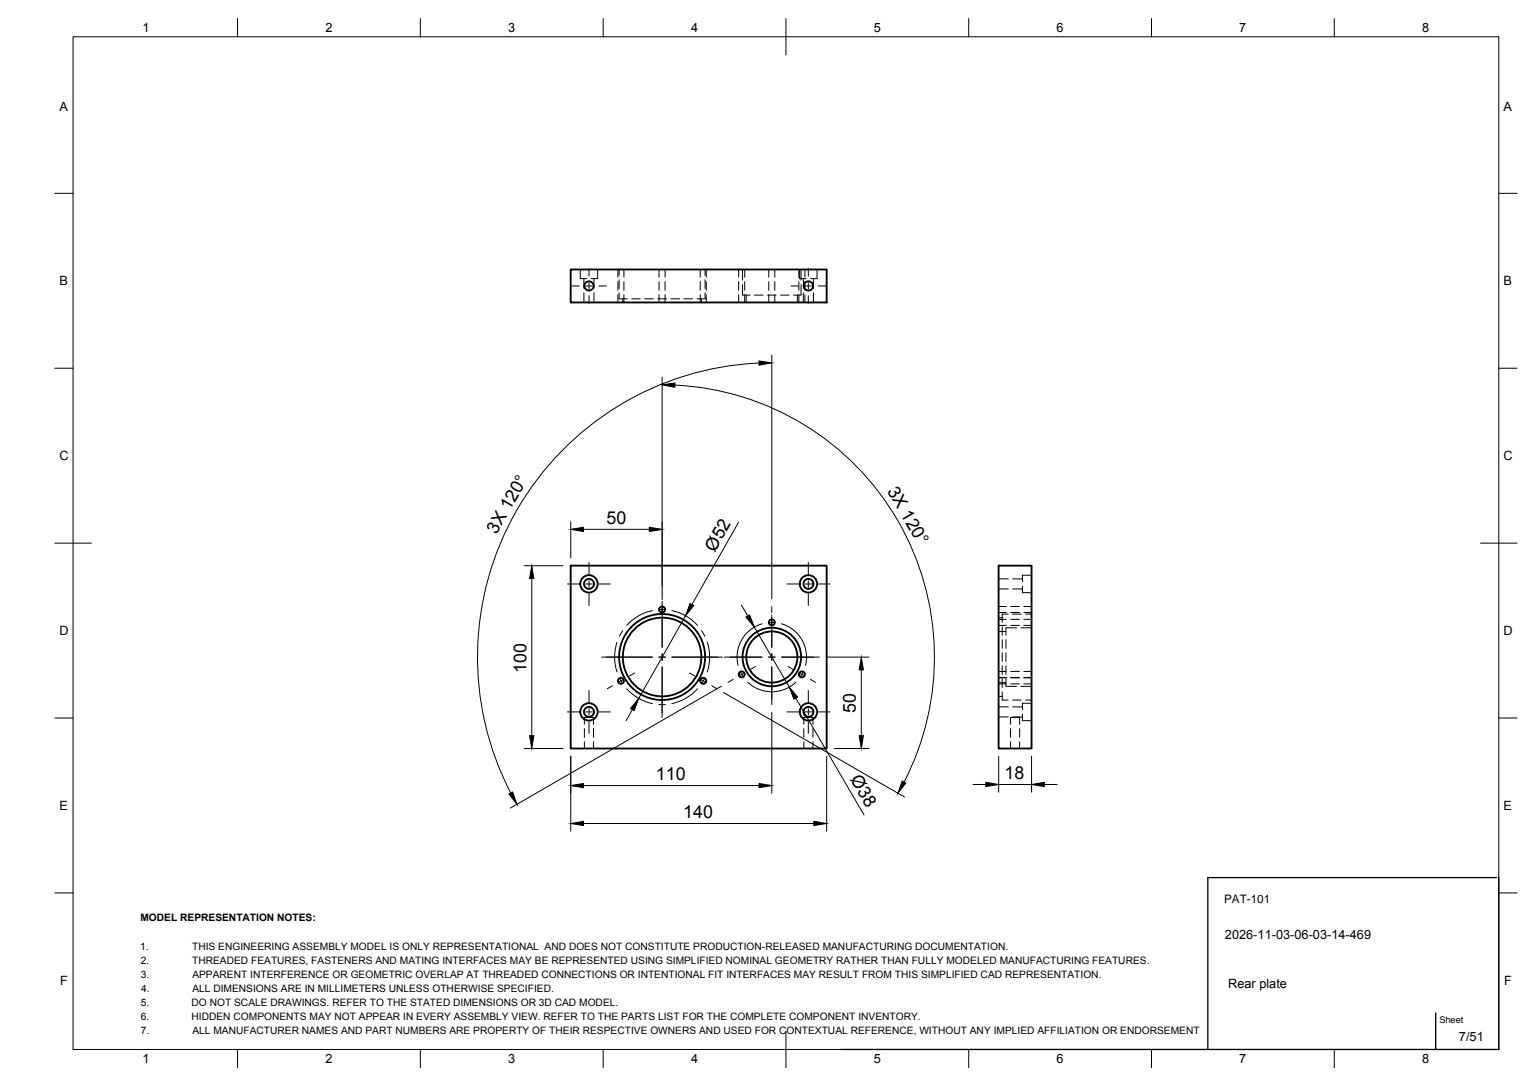
ISO-10303-21;
HEADER;
/* Generated by software containing ST-Developer
 * from STEP Tools, Inc. (www.steptools.com) 
 */

FILE_DESCRIPTION(
/* description */ ('Spur gear reduction stage 2-1 on bearing plates'),
/* implementation_level */ '2;1');

FILE_NAME(
/* name */ 'Rear plate.step',
/* time_stamp */ '2026-10-28T03:22:07-07:00',
/* author */ (''),
/* organization */ (''),
/* preprocessor_version */ 'ST-DEVELOPER v20.2',
/* originating_system */ 'Autodesk Translation Framework v15.17.0.0',
/* authorisation */ '');

FILE_SCHEMA (('AUTOMOTIVE_DESIGN { 1 0 10303 214 3 1 1 }'));
ENDSEC;

DATA;
#10=MECHANICAL_DESIGN_GEOMETRIC_PRESENTATION_REPRESENTATION('',(#949),#53909);
#863=SHAPE_REPRESENTATION_RELATIONSHIP('SRR','None',#54090,#906);
#906=ADVANCED_BREP_SHAPE_REPRESENTATION('',(#1007),#53864);
#949=STYLED_ITEM('',(#54411),#1007);
#1007=MANIFOLD_SOLID_BREP('Body1',#11273);
#1100=FACE_BOUND('',#2243,.T.);
#1101=FACE_BOUND('',#2246,.T.);
#1102=FACE_BOUND('',#2249,.T.);
#1103=FACE_BOUND('',#2252,.T.);
#1104=FACE_BOUND('',#2263,.T.);
#1105=FACE_BOUND('',#2267,.T.);
#1106=FACE_BOUND('',#2270,.T.);
#1107=FACE_BOUND('',#2271,.T.);
#1108=FACE_BOUND('',#2272,.T.);
#1109=FACE_BOUND('',#2273,.T.);
#1110=FACE_BOUND('',#2274,.T.);
#1111=FACE_BOUND('',#2275,.T.);
#1112=FACE_BOUND('',#2276,.T.);
#1113=FACE_BOUND('',#2277,.T.);
#1114=FACE_BOUND('',#2278,.T.);
#1115=FACE_BOUND('',#2279,.T.);
#1116=FACE_BOUND('',#2280,.T.);
#1117=FACE_BOUND('',#2281,.T.);
#1118=FACE_BOUND('',#2284,.T.);
#1119=FACE_BOUND('',#2285,.T.);
#1120=FACE_BOUND('',#2286,.T.);
#1121=FACE_BOUND('',#2287,.T.);
#1122=FACE_BOUND('',#2288,.T.);
#1123=FACE_BOUND('',#2289,.T.);
#1124=FACE_BOUND('',#2290,.T.);
#1125=FACE_BOUND('',#2291,.T.);
#1126=FACE_BOUND('',#2292,.T.);
#1127=FACE_BOUND('',#2293,.T.);
#1128=FACE_BOUND('',#2294,.T.);
#1129=FACE_BOUND('',#2295,.T.);
#1130=FACE_BOUND('',#2299,.T.);
#1131=FACE_BOUND('',#2300,.T.);
#1258=PLANE('',#11924);
#1259=PLANE('',#11929);
#1260=PLANE('',#11934);
#1261=PLANE('',#11939);
#1262=PLANE('',#11952);
#1263=PLANE('',#11956);
#1264=PLANE('',#11960);
#1265=PLANE('',#11967);
#1266=PLANE('',#11971);
#1267=PLANE('',#11972);
#1268=PLANE('',#11973);
#1269=PLANE('',#11974);
#1270=PLANE('',#11975);
#1271=PLANE('',#11976);
#1547=FACE_OUTER_BOUND('',#2235,.T.);
#1548=FACE_OUTER_BOUND('',#2236,.T.);
#1549=FACE_OUTER_BOUND('',#2237,.T.);
#1550=FACE_OUTER_BOUND('',#2238,.T.);
#1551=FACE_OUTER_BOUND('',#2239,.T.);
#1552=FACE_OUTER_BOUND('',#2240,.T.);
#1553=FACE_OUTER_BOUND('',#2241,.T.);
#1554=FACE_OUTER_BOUND('',#2242,.T.);
#1555=FACE_OUTER_BOUND('',#2244,.T.);
#1556=FACE_OUTER_BOUND('',#2245,.T.);
#1557=FACE_OUTER_BOUND('',#2247,.T.);
#1558=FACE_OUTER_BOUND('',#2248,.T.);
#1559=FACE_OUTER_BOUND('',#2250,.T.);
#1560=FACE_OUTER_BOUND('',#2251,.T.);
#1561=FACE_OUTER_BOUND('',#2253,.T.);
#1562=FACE_OUTER_BOUND('',#2254,.T.);
#1563=FACE_OUTER_BOUND('',#2255,.T.);
#1564=FACE_OUTER_BOUND('',#2256,.T.);
#1565=FACE_OUTER_BOUND('',#2257,.T.);
#1566=FACE_OUTER_BOUND('',#2258,.T.);
#1567=FACE_OUTER_BOUND('',#2259,.T.);
#1568=FACE_OUTER_BOUND('',#2260,.T.);
#1569=FACE_OUTER_BOUND('',#2261,.T.);
#1570=FACE_OUTER_BOUND('',#2262,.T.);
#1571=FACE_OUTER_BOUND('',#2264,.T.);
#1572=FACE_OUTER_BOUND('',#2265,.T.);
#1573=FACE_OUTER_BOUND('',#2266,.T.);
#1574=FACE_OUTER_BOUND('',#2268,.T.);
#1575=FACE_OUTER_BOUND('',#2269,.T.);
#1576=FACE_OUTER_BOUND('',#2282,.T.);
#1577=FACE_OUTER_BOUND('',#2283,.T.);
#1578=FACE_OUTER_BOUND('',#2296,.T.);
#1579=FACE_OUTER_BOUND('',#2297,.T.);
#1580=FACE_OUTER_BOUND('',#2298,.T.);
#2235=EDGE_LOOP('',(#7544,#7545,#7546,#7547));
#2236=EDGE_LOOP('',(#7548,#7549,#7550,#7551));
#2237=EDGE_LOOP('',(#7552,#7553,#7554,#7555));
#2238=EDGE_LOOP('',(#7556,#7557,#7558,#7559));
#2239=EDGE_LOOP('',(#7560,#7561,#7562,#7563));
#2240=EDGE_LOOP('',(#7564,#7565,#7566,#7567));
#2241=EDGE_LOOP('',(#7568,#7569,#7570,#7571));
#2242=EDGE_LOOP('',(#7572));
#2243=EDGE_LOOP('',(#7573));
#2244=EDGE_LOOP('',(#7574,#7575,#7576,#7577));
#2245=EDGE_LOOP('',(#7578));
#2246=EDGE_LOOP('',(#7579));
#2247=EDGE_LOOP('',(#7580,#7581,#7582,#7583));
#2248=EDGE_LOOP('',(#7584));
#2249=EDGE_LOOP('',(#7585));
#2250=EDGE_LOOP('',(#7586,#7587,#7588,#7589));
#2251=EDGE_LOOP('',(#7590));
#2252=EDGE_LOOP('',(#7591));
#2253=EDGE_LOOP('',(#7592,#7593,#7594,#7595));
#2254=EDGE_LOOP('',(#7596,#7597,#7598,#7599));
#2255=EDGE_LOOP('',(#7600,#7601,#7602,#7603));
#2256=EDGE_LOOP('',(#7604,#7605,#7606,#7607));
#2257=EDGE_LOOP('',(#7608,#7609,#7610,#7611));
#2258=EDGE_LOOP('',(#7612));
#2259=EDGE_LOOP('',(#7613,#7614,#7615,#7616));
#2260=EDGE_LOOP('',(#7617));
#2261=EDGE_LOOP('',(#7618,#7619,#7620,#7621));
#2262=EDGE_LOOP('',(#7622));
#2263=EDGE_LOOP('',(#7623));
#2264=EDGE_LOOP('',(#7624,#7625,#7626,#7627));
#2265=EDGE_LOOP('',(#7628,#7629,#7630,#7631));
#2266=EDGE_LOOP('',(#7632));
#2267=EDGE_LOOP('',(#7633));
#2268=EDGE_LOOP('',(#7634,#7635,#7636,#7637));
#2269=EDGE_LOOP('',(#7638,#7639,#7640,#7641));
#2270=EDGE_LOOP('',(#7642));
#2271=EDGE_LOOP('',(#7643));
#2272=EDGE_LOOP('',(#7644));
#2273=EDGE_LOOP('',(#7645));
#2274=EDGE_LOOP('',(#7646));
#2275=EDGE_LOOP('',(#7647));
#2276=EDGE_LOOP('',(#7648));
#2277=EDGE_LOOP('',(#7649));
#2278=EDGE_LOOP('',(#7650));
#2279=EDGE_LOOP('',(#7651));
#2280=EDGE_LOOP('',(#7652));
#2281=EDGE_LOOP('',(#7653));
#2282=EDGE_LOOP('',(#7654,#7655,#7656,#7657));
#2283=EDGE_LOOP('',(#7658,#7659,#7660,#7661));
#2284=EDGE_LOOP('',(#7662));
#2285=EDGE_LOOP('',(#7663));
#2286=EDGE_LOOP('',(#7664));
#2287=EDGE_LOOP('',(#7665));
#2288=EDGE_LOOP('',(#7666));
#2289=EDGE_LOOP('',(#7667));
#2290=EDGE_LOOP('',(#7668));
#2291=EDGE_LOOP('',(#7669));
#2292=EDGE_LOOP('',(#7670));
#2293=EDGE_LOOP('',(#7671));
#2294=EDGE_LOOP('',(#7672));
#2295=EDGE_LOOP('',(#7673));
#2296=EDGE_LOOP('',(#7674,#7675,#7676,#7677));
#2297=EDGE_LOOP('',(#7678,#7679,#7680,#7681));
#2298=EDGE_LOOP('',(#7682,#7683,#7684,#7685));
#2299=EDGE_LOOP('',(#7686));
#2300=EDGE_LOOP('',(#7687));
#3025=LINE('',#16188,#3666);
#3026=LINE('',#16194,#3667);
#3027=LINE('',#16200,#3668);
#3028=LINE('',#16206,#3669);
#3029=LINE('',#16212,#3670);
#3030=LINE('',#16218,#3671);
#3031=LINE('',#16224,#3672);
#3032=LINE('',#16233,#3673);
#3033=LINE('',#16242,#3674);
#3034=LINE('',#16251,#3675);
#3035=LINE('',#16259,#3676);
#3036=LINE('',#16263,#3677);
#3037=LINE('',#16267,#3678);
#3038=LINE('',#16271,#3679);
#3039=LINE('',#16276,#3680);
#3040=LINE('',#16283,#3681);
#3041=LINE('',#16290,#3682);
#3042=LINE('',#16298,#3683);
#3043=LINE('',#16303,#3684);
#3044=LINE('',#16311,#3685);
#3045=LINE('',#16315,#3686);
#3046=LINE('',#16317,#3687);
#3047=LINE('',#16319,#3688);
#3048=LINE('',#16320,#3689);
#3049=LINE('',#16323,#3690);
#3050=LINE('',#16325,#3691);
#3051=LINE('',#16326,#3692);
#3052=LINE('',#16329,#3693);
#3053=LINE('',#16331,#3694);
#3054=LINE('',#16332,#3695);
#3055=LINE('',#16334,#3696);
#3056=LINE('',#16335,#3697);
#3666=VECTOR('',#13228,0.165);
#3667=VECTOR('',#13235,0.165);
#3668=VECTOR('',#13242,0.164999999999999);
#3669=VECTOR('',#13249,0.165);
#3670=VECTOR('',#13256,0.165);
#3671=VECTOR('',#13263,0.165);
#3672=VECTOR('',#13270,0.475);
#3673=VECTOR('',#13281,0.475);
#3674=VECTOR('',#13292,0.475);
#3675=VECTOR('',#13303,0.475);
#3676=VECTOR('',#13314,0.275);
#3677=VECTOR('',#13319,0.275);
#3678=VECTOR('',#13324,0.275);
#3679=VECTOR('',#13329,0.275);
#3680=VECTOR('',#13334,0.25);
#3681=VECTOR('',#13343,0.25);
#3682=VECTOR('',#13352,2.35);
#3683=VECTOR('',#13363,2.15);
#3684=VECTOR('',#13368,1.6);
#3685=VECTOR('',#13379,1.4);
#3686=VECTOR('',#13382,1.);
#3687=VECTOR('',#13383,1.);
#3688=VECTOR('',#13384,1.);
#3689=VECTOR('',#13385,1.);
#3690=VECTOR('',#13388,1.);
#3691=VECTOR('',#13389,1.);
#3692=VECTOR('',#13390,1.);
#3693=VECTOR('',#13393,1.);
#3694=VECTOR('',#13394,1.);
#3695=VECTOR('',#13395,1.);
#3696=VECTOR('',#13398,1.);
#3697=VECTOR('',#13399,1.);
#4307=CIRCLE('',#11904,0.165);
#4308=CIRCLE('',#11905,0.165);
#4309=CIRCLE('',#11907,0.165);
#4310=CIRCLE('',#11908,0.165);
#4311=CIRCLE('',#11910,0.164999999999999);
#4312=CIRCLE('',#11911,0.164999999999999);
#4313=CIRCLE('',#11913,0.165);
#4314=CIRCLE('',#11914,0.165);
#4315=CIRCLE('',#11916,0.165);
#4316=CIRCLE('',#11917,0.165);
#4317=CIRCLE('',#11919,0.165);
#4318=CIRCLE('',#11920,0.165);
#4319=CIRCLE('',#11922,0.475);
#4320=CIRCLE('',#11923,0.475);
#4321=CIRCLE('',#11925,0.275);
#4322=CIRCLE('',#11927,0.475);
#4323=CIRCLE('',#11928,0.475);
#4324=CIRCLE('',#11930,0.275);
#4325=CIRCLE('',#11932,0.475);
#4326=CIRCLE('',#11933,0.475);
#4327=CIRCLE('',#11935,0.275);
#4328=CIRCLE('',#11937,0.475);
#4329=CIRCLE('',#11938,0.475);
#4330=CIRCLE('',#11940,0.275);
#4331=CIRCLE('',#11942,0.275);
#4332=CIRCLE('',#11944,0.275);
#4333=CIRCLE('',#11946,0.275);
#4334=CIRCLE('',#11948,0.275);
#4335=CIRCLE('',#11950,0.25);
#4336=CIRCLE('',#11951,0.25);
#4337=CIRCLE('',#11954,0.25);
#4338=CIRCLE('',#11955,0.25);
#4339=CIRCLE('',#11958,2.35);
#4340=CIRCLE('',#11959,2.35);
#4341=CIRCLE('',#11961,2.15);
#4342=CIRCLE('',#11963,2.15);
#4343=CIRCLE('',#11965,1.6);
#4344=CIRCLE('',#11966,1.6);
#4345=CIRCLE('',#11968,1.4);
#4346=CIRCLE('',#11970,1.4);
#4848=VERTEX_POINT('',#16185);
#4849=VERTEX_POINT('',#16187);
#4850=VERTEX_POINT('',#16191);
#4851=VERTEX_POINT('',#16193);
#4852=VERTEX_POINT('',#16197);
#4853=VERTEX_POINT('',#16199);
#4854=VERTEX_POINT('',#16203);
#4855=VERTEX_POINT('',#16205);
#4856=VERTEX_POINT('',#16209);
#4857=VERTEX_POINT('',#16211);
#4858=VERTEX_POINT('',#16215);
#4859=VERTEX_POINT('',#16217);
#4860=VERTEX_POINT('',#16221);
#4861=VERTEX_POINT('',#16223);
#4862=VERTEX_POINT('',#16227);
#4863=VERTEX_POINT('',#16230);
#4864=VERTEX_POINT('',#16232);
#4865=VERTEX_POINT('',#16236);
#4866=VERTEX_POINT('',#16239);
#4867=VERTEX_POINT('',#16241);
#4868=VERTEX_POINT('',#16245);
#4869=VERTEX_POINT('',#16248);
#4870=VERTEX_POINT('',#16250);
#4871=VERTEX_POINT('',#16254);
#4872=VERTEX_POINT('',#16257);
#4873=VERTEX_POINT('',#16261);
#4874=VERTEX_POINT('',#16265);
#4875=VERTEX_POINT('',#16269);
#4876=VERTEX_POINT('',#16273);
#4877=VERTEX_POINT('',#16275);
#4878=VERTEX_POINT('',#16280);
#4879=VERTEX_POINT('',#16282);
#4880=VERTEX_POINT('',#16287);
#4881=VERTEX_POINT('',#16289);
#4882=VERTEX_POINT('',#16293);
#4883=VERTEX_POINT('',#16296);
#4884=VERTEX_POINT('',#16300);
#4885=VERTEX_POINT('',#16302);
#4886=VERTEX_POINT('',#16306);
#4887=VERTEX_POINT('',#16309);
#4888=VERTEX_POINT('',#16313);
#4889=VERTEX_POINT('',#16314);
#4890=VERTEX_POINT('',#16316);
#4891=VERTEX_POINT('',#16318);
#4892=VERTEX_POINT('',#16322);
#4893=VERTEX_POINT('',#16324);
#4894=VERTEX_POINT('',#16328);
#4895=VERTEX_POINT('',#16330);
#5914=EDGE_CURVE('',#4848,#4848,#4307,.T.);
#5915=EDGE_CURVE('',#4848,#4849,#3025,.T.);
#5916=EDGE_CURVE('',#4849,#4849,#4308,.T.);
#5917=EDGE_CURVE('',#4850,#4850,#4309,.T.);
#5918=EDGE_CURVE('',#4850,#4851,#3026,.T.);
#5919=EDGE_CURVE('',#4851,#4851,#4310,.T.);
#5920=EDGE_CURVE('',#4852,#4852,#4311,.T.);
#5921=EDGE_CURVE('',#4852,#4853,#3027,.T.);
#5922=EDGE_CURVE('',#4853,#4853,#4312,.T.);
#5923=EDGE_CURVE('',#4854,#4854,#4313,.T.);
#5924=EDGE_CURVE('',#4854,#4855,#3028,.T.);
#5925=EDGE_CURVE('',#4855,#4855,#4314,.T.);
#5926=EDGE_CURVE('',#4856,#4856,#4315,.T.);
#5927=EDGE_CURVE('',#4856,#4857,#3029,.T.);
#5928=EDGE_CURVE('',#4857,#4857,#4316,.T.);
#5929=EDGE_CURVE('',#4858,#4858,#4317,.T.);
#5930=EDGE_CURVE('',#4858,#4859,#3030,.T.);
#5931=EDGE_CURVE('',#4859,#4859,#4318,.T.);
#5932=EDGE_CURVE('',#4860,#4860,#4319,.T.);
#5933=EDGE_CURVE('',#4860,#4861,#3031,.T.);
#5934=EDGE_CURVE('',#4861,#4861,#4320,.T.);
#5935=EDGE_CURVE('',#4862,#4862,#4321,.T.);
#5936=EDGE_CURVE('',#4863,#4863,#4322,.T.);
#5937=EDGE_CURVE('',#4863,#4864,#3032,.T.);
#5938=EDGE_CURVE('',#4864,#4864,#4323,.T.);
#5939=EDGE_CURVE('',#4865,#4865,#4324,.T.);
#5940=EDGE_CURVE('',#4866,#4866,#4325,.T.);
#5941=EDGE_CURVE('',#4866,#4867,#3033,.T.);
#5942=EDGE_CURVE('',#4867,#4867,#4326,.T.);
#5943=EDGE_CURVE('',#4868,#4868,#4327,.T.);
#5944=EDGE_CURVE('',#4869,#4869,#4328,.T.);
#5945=EDGE_CURVE('',#4869,#4870,#3034,.T.);
#5946=EDGE_CURVE('',#4870,#4870,#4329,.T.);
#5947=EDGE_CURVE('',#4871,#4871,#4330,.T.);
#5948=EDGE_CURVE('',#4872,#4872,#4331,.T.);
#5949=EDGE_CURVE('',#4872,#4862,#3035,.T.);
#5950=EDGE_CURVE('',#4873,#4873,#4332,.T.);
#5951=EDGE_CURVE('',#4873,#4865,#3036,.T.);
#5952=EDGE_CURVE('',#4874,#4874,#4333,.T.);
#5953=EDGE_CURVE('',#4874,#4868,#3037,.T.);
#5954=EDGE_CURVE('',#4875,#4875,#4334,.T.);
#5955=EDGE_CURVE('',#4875,#4871,#3038,.T.);
#5956=EDGE_CURVE('',#4876,#4876,#4335,.T.);
#5957=EDGE_CURVE('',#4876,#4877,#3039,.T.);
#5958=EDGE_CURVE('',#4877,#4877,#4336,.T.);
#5959=EDGE_CURVE('',#4878,#4878,#4337,.T.);
#5960=EDGE_CURVE('',#4878,#4879,#3040,.T.);
#5961=EDGE_CURVE('',#4879,#4879,#4338,.T.);
#5962=EDGE_CURVE('',#4880,#4880,#4339,.T.);
#5963=EDGE_CURVE('',#4880,#4881,#3041,.T.);
#5964=EDGE_CURVE('',#4881,#4881,#4340,.T.);
#5965=EDGE_CURVE('',#4882,#4882,#4341,.T.);
#5966=EDGE_CURVE('',#4883,#4883,#4342,.T.);
#5967=EDGE_CURVE('',#4883,#4882,#3042,.T.);
#5968=EDGE_CURVE('',#4884,#4884,#4343,.T.);
#5969=EDGE_CURVE('',#4884,#4885,#3043,.T.);
#5970=EDGE_CURVE('',#4885,#4885,#4344,.T.);
#5971=EDGE_CURVE('',#4886,#4886,#4345,.T.);
#5972=EDGE_CURVE('',#4887,#4887,#4346,.T.);
#5973=EDGE_CURVE('',#4887,#4886,#3044,.T.);
#5974=EDGE_CURVE('',#4888,#4889,#3045,.T.);
#5975=EDGE_CURVE('',#4889,#4890,#3046,.T.);
#5976=EDGE_CURVE('',#4891,#4890,#3047,.T.);
#5977=EDGE_CURVE('',#4888,#4891,#3048,.T.);
#5978=EDGE_CURVE('',#4892,#4888,#3049,.T.);
#5979=EDGE_CURVE('',#4893,#4891,#3050,.T.);
#5980=EDGE_CURVE('',#4892,#4893,#3051,.T.);
#5981=EDGE_CURVE('',#4894,#4892,#3052,.T.);
#5982=EDGE_CURVE('',#4895,#4893,#3053,.T.);
#5983=EDGE_CURVE('',#4894,#4895,#3054,.T.);
#5984=EDGE_CURVE('',#4889,#4894,#3055,.T.);
#5985=EDGE_CURVE('',#4890,#4895,#3056,.T.);
#7544=ORIENTED_EDGE('',*,*,#5914,.F.);
#7545=ORIENTED_EDGE('',*,*,#5915,.T.);
#7546=ORIENTED_EDGE('',*,*,#5916,.F.);
#7547=ORIENTED_EDGE('',*,*,#5915,.F.);
#7548=ORIENTED_EDGE('',*,*,#5917,.F.);
#7549=ORIENTED_EDGE('',*,*,#5918,.T.);
#7550=ORIENTED_EDGE('',*,*,#5919,.F.);
#7551=ORIENTED_EDGE('',*,*,#5918,.F.);
#7552=ORIENTED_EDGE('',*,*,#5920,.F.);
#7553=ORIENTED_EDGE('',*,*,#5921,.T.);
#7554=ORIENTED_EDGE('',*,*,#5922,.F.);
#7555=ORIENTED_EDGE('',*,*,#5921,.F.);
#7556=ORIENTED_EDGE('',*,*,#5923,.F.);
#7557=ORIENTED_EDGE('',*,*,#5924,.T.);
#7558=ORIENTED_EDGE('',*,*,#5925,.F.);
#7559=ORIENTED_EDGE('',*,*,#5924,.F.);
#7560=ORIENTED_EDGE('',*,*,#5926,.F.);
#7561=ORIENTED_EDGE('',*,*,#5927,.T.);
#7562=ORIENTED_EDGE('',*,*,#5928,.F.);
#7563=ORIENTED_EDGE('',*,*,#5927,.F.);
#7564=ORIENTED_EDGE('',*,*,#5929,.F.);
#7565=ORIENTED_EDGE('',*,*,#5930,.T.);
#7566=ORIENTED_EDGE('',*,*,#5931,.F.);
#7567=ORIENTED_EDGE('',*,*,#5930,.F.);
#7568=ORIENTED_EDGE('',*,*,#5932,.F.);
#7569=ORIENTED_EDGE('',*,*,#5933,.T.);
#7570=ORIENTED_EDGE('',*,*,#5934,.F.);
#7571=ORIENTED_EDGE('',*,*,#5933,.F.);
#7572=ORIENTED_EDGE('',*,*,#5932,.T.);
#7573=ORIENTED_EDGE('',*,*,#5935,.F.);
#7574=ORIENTED_EDGE('',*,*,#5936,.F.);
#7575=ORIENTED_EDGE('',*,*,#5937,.T.);
#7576=ORIENTED_EDGE('',*,*,#5938,.F.);
#7577=ORIENTED_EDGE('',*,*,#5937,.F.);
#7578=ORIENTED_EDGE('',*,*,#5936,.T.);
#7579=ORIENTED_EDGE('',*,*,#5939,.F.);
#7580=ORIENTED_EDGE('',*,*,#5940,.F.);
#7581=ORIENTED_EDGE('',*,*,#5941,.T.);
#7582=ORIENTED_EDGE('',*,*,#5942,.F.);
#7583=ORIENTED_EDGE('',*,*,#5941,.F.);
#7584=ORIENTED_EDGE('',*,*,#5940,.T.);
#7585=ORIENTED_EDGE('',*,*,#5943,.F.);
#7586=ORIENTED_EDGE('',*,*,#5944,.F.);
#7587=ORIENTED_EDGE('',*,*,#5945,.T.);
#7588=ORIENTED_EDGE('',*,*,#5946,.F.);
#7589=ORIENTED_EDGE('',*,*,#5945,.F.);
#7590=ORIENTED_EDGE('',*,*,#5944,.T.);
#7591=ORIENTED_EDGE('',*,*,#5947,.F.);
#7592=ORIENTED_EDGE('',*,*,#5948,.F.);
#7593=ORIENTED_EDGE('',*,*,#5949,.T.);
#7594=ORIENTED_EDGE('',*,*,#5935,.T.);
#7595=ORIENTED_EDGE('',*,*,#5949,.F.);
#7596=ORIENTED_EDGE('',*,*,#5950,.F.);
#7597=ORIENTED_EDGE('',*,*,#5951,.T.);
#7598=ORIENTED_EDGE('',*,*,#5939,.T.);
#7599=ORIENTED_EDGE('',*,*,#5951,.F.);
#7600=ORIENTED_EDGE('',*,*,#5952,.F.);
#7601=ORIENTED_EDGE('',*,*,#5953,.T.);
#7602=ORIENTED_EDGE('',*,*,#5943,.T.);
#7603=ORIENTED_EDGE('',*,*,#5953,.F.);
#7604=ORIENTED_EDGE('',*,*,#5954,.F.);
#7605=ORIENTED_EDGE('',*,*,#5955,.T.);
#7606=ORIENTED_EDGE('',*,*,#5947,.T.);
#7607=ORIENTED_EDGE('',*,*,#5955,.F.);
#7608=ORIENTED_EDGE('',*,*,#5956,.F.);
#7609=ORIENTED_EDGE('',*,*,#5957,.T.);
#7610=ORIENTED_EDGE('',*,*,#5958,.T.);
#7611=ORIENTED_EDGE('',*,*,#5957,.F.);
#7612=ORIENTED_EDGE('',*,*,#5958,.F.);
#7613=ORIENTED_EDGE('',*,*,#5959,.F.);
#7614=ORIENTED_EDGE('',*,*,#5960,.T.);
#7615=ORIENTED_EDGE('',*,*,#5961,.T.);
#7616=ORIENTED_EDGE('',*,*,#5960,.F.);
#7617=ORIENTED_EDGE('',*,*,#5961,.F.);
#7618=ORIENTED_EDGE('',*,*,#5962,.F.);
#7619=ORIENTED_EDGE('',*,*,#5963,.T.);
#7620=ORIENTED_EDGE('',*,*,#5964,.F.);
#7621=ORIENTED_EDGE('',*,*,#5963,.F.);
#7622=ORIENTED_EDGE('',*,*,#5962,.T.);
#7623=ORIENTED_EDGE('',*,*,#5965,.F.);
#7624=ORIENTED_EDGE('',*,*,#5966,.F.);
#7625=ORIENTED_EDGE('',*,*,#5967,.T.);
#7626=ORIENTED_EDGE('',*,*,#5965,.T.);
#7627=ORIENTED_EDGE('',*,*,#5967,.F.);
#7628=ORIENTED_EDGE('',*,*,#5968,.F.);
#7629=ORIENTED_EDGE('',*,*,#5969,.T.);
#7630=ORIENTED_EDGE('',*,*,#5970,.F.);
#7631=ORIENTED_EDGE('',*,*,#5969,.F.);
#7632=ORIENTED_EDGE('',*,*,#5968,.T.);
#7633=ORIENTED_EDGE('',*,*,#5971,.F.);
#7634=ORIENTED_EDGE('',*,*,#5972,.F.);
#7635=ORIENTED_EDGE('',*,*,#5973,.T.);
#7636=ORIENTED_EDGE('',*,*,#5971,.T.);
#7637=ORIENTED_EDGE('',*,*,#5973,.F.);
#7638=ORIENTED_EDGE('',*,*,#5974,.T.);
#7639=ORIENTED_EDGE('',*,*,#5975,.T.);
#7640=ORIENTED_EDGE('',*,*,#5976,.F.);
#7641=ORIENTED_EDGE('',*,*,#5977,.F.);
#7642=ORIENTED_EDGE('',*,*,#5925,.T.);
#7643=ORIENTED_EDGE('',*,*,#5928,.T.);
#7644=ORIENTED_EDGE('',*,*,#5931,.T.);
#7645=ORIENTED_EDGE('',*,*,#5964,.T.);
#7646=ORIENTED_EDGE('',*,*,#5970,.T.);
#7647=ORIENTED_EDGE('',*,*,#5946,.T.);
#7648=ORIENTED_EDGE('',*,*,#5942,.T.);
#7649=ORIENTED_EDGE('',*,*,#5938,.T.);
#7650=ORIENTED_EDGE('',*,*,#5934,.T.);
#7651=ORIENTED_EDGE('',*,*,#5922,.T.);
#7652=ORIENTED_EDGE('',*,*,#5919,.T.);
#7653=ORIENTED_EDGE('',*,*,#5916,.T.);
#7654=ORIENTED_EDGE('',*,*,#5978,.T.);
#7655=ORIENTED_EDGE('',*,*,#5977,.T.);
#7656=ORIENTED_EDGE('',*,*,#5979,.F.);
#7657=ORIENTED_EDGE('',*,*,#5980,.F.);
#7658=ORIENTED_EDGE('',*,*,#5981,.T.);
#7659=ORIENTED_EDGE('',*,*,#5980,.T.);
#7660=ORIENTED_EDGE('',*,*,#5982,.F.);
#7661=ORIENTED_EDGE('',*,*,#5983,.F.);
#7662=ORIENTED_EDGE('',*,*,#5923,.T.);
#7663=ORIENTED_EDGE('',*,*,#5926,.T.);
#7664=ORIENTED_EDGE('',*,*,#5929,.T.);
#7665=ORIENTED_EDGE('',*,*,#5972,.T.);
#7666=ORIENTED_EDGE('',*,*,#5966,.T.);
#7667=ORIENTED_EDGE('',*,*,#5954,.T.);
#7668=ORIENTED_EDGE('',*,*,#5952,.T.);
#7669=ORIENTED_EDGE('',*,*,#5950,.T.);
#7670=ORIENTED_EDGE('',*,*,#5948,.T.);
#7671=ORIENTED_EDGE('',*,*,#5920,.T.);
#7672=ORIENTED_EDGE('',*,*,#5917,.T.);
#7673=ORIENTED_EDGE('',*,*,#5914,.T.);
#7674=ORIENTED_EDGE('',*,*,#5984,.T.);
#7675=ORIENTED_EDGE('',*,*,#5983,.T.);
#7676=ORIENTED_EDGE('',*,*,#5985,.F.);
#7677=ORIENTED_EDGE('',*,*,#5975,.F.);
#7678=ORIENTED_EDGE('',*,*,#5985,.T.);
#7679=ORIENTED_EDGE('',*,*,#5982,.T.);
#7680=ORIENTED_EDGE('',*,*,#5979,.T.);
#7681=ORIENTED_EDGE('',*,*,#5976,.T.);
#7682=ORIENTED_EDGE('',*,*,#5984,.F.);
#7683=ORIENTED_EDGE('',*,*,#5974,.F.);
#7684=ORIENTED_EDGE('',*,*,#5978,.F.);
#7685=ORIENTED_EDGE('',*,*,#5981,.F.);
#7686=ORIENTED_EDGE('',*,*,#5956,.T.);
#7687=ORIENTED_EDGE('',*,*,#5959,.T.);
#10444=CYLINDRICAL_SURFACE('',#11903,0.165);
#10445=CYLINDRICAL_SURFACE('',#11906,0.165);
#10446=CYLINDRICAL_SURFACE('',#11909,0.164999999999999);
#10447=CYLINDRICAL_SURFACE('',#11912,0.165);
#10448=CYLINDRICAL_SURFACE('',#11915,0.165);
#10449=CYLINDRICAL_SURFACE('',#11918,0.165);
#10450=CYLINDRICAL_SURFACE('',#11921,0.475);
#10451=CYLINDRICAL_SURFACE('',#11926,0.475);
#10452=CYLINDRICAL_SURFACE('',#11931,0.475);
#10453=CYLINDRICAL_SURFACE('',#11936,0.475);
#10454=CYLINDRICAL_SURFACE('',#11941,0.275);
#10455=CYLINDRICAL_SURFACE('',#11943,0.275);
#10456=CYLINDRICAL_SURFACE('',#11945,0.275);
#10457=CYLINDRICAL_SURFACE('',#11947,0.275);
#10458=CYLINDRICAL_SURFACE('',#11949,0.25);
#10459=CYLINDRICAL_SURFACE('',#11953,0.25);
#10460=CYLINDRICAL_SURFACE('',#11957,2.35);
#10461=CYLINDRICAL_SURFACE('',#11962,2.15);
#10462=CYLINDRICAL_SURFACE('',#11964,1.6);
#10463=CYLINDRICAL_SURFACE('',#11969,1.4);
#10667=ADVANCED_FACE('',(#1547),#10444,.F.);
#10668=ADVANCED_FACE('',(#1548),#10445,.F.);
#10669=ADVANCED_FACE('',(#1549),#10446,.F.);
#10670=ADVANCED_FACE('',(#1550),#10447,.F.);
#10671=ADVANCED_FACE('',(#1551),#10448,.F.);
#10672=ADVANCED_FACE('',(#1552),#10449,.F.);
#10673=ADVANCED_FACE('',(#1553),#10450,.F.);
#10674=ADVANCED_FACE('',(#1554,#1100),#1258,.T.);
#10675=ADVANCED_FACE('',(#1555),#10451,.F.);
#10676=ADVANCED_FACE('',(#1556,#1101),#1259,.T.);
#10677=ADVANCED_FACE('',(#1557),#10452,.F.);
#10678=ADVANCED_FACE('',(#1558,#1102),#1260,.T.);
#10679=ADVANCED_FACE('',(#1559),#10453,.F.);
#10680=ADVANCED_FACE('',(#1560,#1103),#1261,.T.);
#10681=ADVANCED_FACE('',(#1561),#10454,.F.);
#10682=ADVANCED_FACE('',(#1562),#10455,.F.);
#10683=ADVANCED_FACE('',(#1563),#10456,.F.);
#10684=ADVANCED_FACE('',(#1564),#10457,.F.);
#10685=ADVANCED_FACE('',(#1565),#10458,.F.);
#10686=ADVANCED_FACE('',(#1566),#1262,.F.);
#10687=ADVANCED_FACE('',(#1567),#10459,.F.);
#10688=ADVANCED_FACE('',(#1568),#1263,.F.);
#10689=ADVANCED_FACE('',(#1569),#10460,.F.);
#10690=ADVANCED_FACE('',(#1570,#1104),#1264,.T.);
#10691=ADVANCED_FACE('',(#1571),#10461,.F.);
#10692=ADVANCED_FACE('',(#1572),#10462,.F.);
#10693=ADVANCED_FACE('',(#1573,#1105),#1265,.T.);
#10694=ADVANCED_FACE('',(#1574),#10463,.F.);
#10695=ADVANCED_FACE('',(#1575,#1106,#1107,#1108,#1109,#1110,#1111,#1112,
#1113,#1114,#1115,#1116,#1117),#1266,.T.);
#10696=ADVANCED_FACE('',(#1576),#1267,.T.);
#10697=ADVANCED_FACE('',(#1577,#1118,#1119,#1120,#1121,#1122,#1123,#1124,
#1125,#1126,#1127,#1128,#1129),#1268,.T.);
#10698=ADVANCED_FACE('',(#1578),#1269,.T.);
#10699=ADVANCED_FACE('',(#1579),#1270,.T.);
#10700=ADVANCED_FACE('',(#1580,#1130,#1131),#1271,.F.);
#11273=CLOSED_SHELL('',(#10667,#10668,#10669,#10670,#10671,#10672,#10673,
#10674,#10675,#10676,#10677,#10678,#10679,#10680,#10681,#10682,#10683,#10684,
#10685,#10686,#10687,#10688,#10689,#10690,#10691,#10692,#10693,#10694,#10695,
#10696,#10697,#10698,#10699,#10700));
#11902=AXIS2_PLACEMENT_3D('',#16183,#13222,#13223);
#11903=AXIS2_PLACEMENT_3D('',#16184,#13224,#13225);
#11904=AXIS2_PLACEMENT_3D('',#16186,#13226,#13227);
#11905=AXIS2_PLACEMENT_3D('',#16189,#13229,#13230);
#11906=AXIS2_PLACEMENT_3D('',#16190,#13231,#13232);
#11907=AXIS2_PLACEMENT_3D('',#16192,#13233,#13234);
#11908=AXIS2_PLACEMENT_3D('',#16195,#13236,#13237);
#11909=AXIS2_PLACEMENT_3D('',#16196,#13238,#13239);
#11910=AXIS2_PLACEMENT_3D('',#16198,#13240,#13241);
#11911=AXIS2_PLACEMENT_3D('',#16201,#13243,#13244);
#11912=AXIS2_PLACEMENT_3D('',#16202,#13245,#13246);
#11913=AXIS2_PLACEMENT_3D('',#16204,#13247,#13248);
#11914=AXIS2_PLACEMENT_3D('',#16207,#13250,#13251);
#11915=AXIS2_PLACEMENT_3D('',#16208,#13252,#13253);
#11916=AXIS2_PLACEMENT_3D('',#16210,#13254,#13255);
#11917=AXIS2_PLACEMENT_3D('',#16213,#13257,#13258);
#11918=AXIS2_PLACEMENT_3D('',#16214,#13259,#13260);
#11919=AXIS2_PLACEMENT_3D('',#16216,#13261,#13262);
#11920=AXIS2_PLACEMENT_3D('',#16219,#13264,#13265);
#11921=AXIS2_PLACEMENT_3D('',#16220,#13266,#13267);
#11922=AXIS2_PLACEMENT_3D('',#16222,#13268,#13269);
#11923=AXIS2_PLACEMENT_3D('',#16225,#13271,#13272);
#11924=AXIS2_PLACEMENT_3D('',#16226,#13273,#13274);
#11925=AXIS2_PLACEMENT_3D('',#16228,#13275,#13276);
#11926=AXIS2_PLACEMENT_3D('',#16229,#13277,#13278);
#11927=AXIS2_PLACEMENT_3D('',#16231,#13279,#13280);
#11928=AXIS2_PLACEMENT_3D('',#16234,#13282,#13283);
#11929=AXIS2_PLACEMENT_3D('',#16235,#13284,#13285);
#11930=AXIS2_PLACEMENT_3D('',#16237,#13286,#13287);
#11931=AXIS2_PLACEMENT_3D('',#16238,#13288,#13289);
#11932=AXIS2_PLACEMENT_3D('',#16240,#13290,#13291);
#11933=AXIS2_PLACEMENT_3D('',#16243,#13293,#13294);
#11934=AXIS2_PLACEMENT_3D('',#16244,#13295,#13296);
#11935=AXIS2_PLACEMENT_3D('',#16246,#13297,#13298);
#11936=AXIS2_PLACEMENT_3D('',#16247,#13299,#13300);
#11937=AXIS2_PLACEMENT_3D('',#16249,#13301,#13302);
#11938=AXIS2_PLACEMENT_3D('',#16252,#13304,#13305);
#11939=AXIS2_PLACEMENT_3D('',#16253,#13306,#13307);
#11940=AXIS2_PLACEMENT_3D('',#16255,#13308,#13309);
#11941=AXIS2_PLACEMENT_3D('',#16256,#13310,#13311);
#11942=AXIS2_PLACEMENT_3D('',#16258,#13312,#13313);
#11943=AXIS2_PLACEMENT_3D('',#16260,#13315,#13316);
#11944=AXIS2_PLACEMENT_3D('',#16262,#13317,#13318);
#11945=AXIS2_PLACEMENT_3D('',#16264,#13320,#13321);
#11946=AXIS2_PLACEMENT_3D('',#16266,#13322,#13323);
#11947=AXIS2_PLACEMENT_3D('',#16268,#13325,#13326);
#11948=AXIS2_PLACEMENT_3D('',#16270,#13327,#13328);
#11949=AXIS2_PLACEMENT_3D('',#16272,#13330,#13331);
#11950=AXIS2_PLACEMENT_3D('',#16274,#13332,#13333);
#11951=AXIS2_PLACEMENT_3D('',#16277,#13335,#13336);
#11952=AXIS2_PLACEMENT_3D('',#16278,#13337,#13338);
#11953=AXIS2_PLACEMENT_3D('',#16279,#13339,#13340);
#11954=AXIS2_PLACEMENT_3D('',#16281,#13341,#13342);
#11955=AXIS2_PLACEMENT_3D('',#16284,#13344,#13345);
#11956=AXIS2_PLACEMENT_3D('',#16285,#13346,#13347);
#11957=AXIS2_PLACEMENT_3D('',#16286,#13348,#13349);
#11958=AXIS2_PLACEMENT_3D('',#16288,#13350,#13351);
#11959=AXIS2_PLACEMENT_3D('',#16291,#13353,#13354);
#11960=AXIS2_PLACEMENT_3D('',#16292,#13355,#13356);
#11961=AXIS2_PLACEMENT_3D('',#16294,#13357,#13358);
#11962=AXIS2_PLACEMENT_3D('',#16295,#13359,#13360);
#11963=AXIS2_PLACEMENT_3D('',#16297,#13361,#13362);
#11964=AXIS2_PLACEMENT_3D('',#16299,#13364,#13365);
#11965=AXIS2_PLACEMENT_3D('',#16301,#13366,#13367);
#11966=AXIS2_PLACEMENT_3D('',#16304,#13369,#13370);
#11967=AXIS2_PLACEMENT_3D('',#16305,#13371,#13372);
#11968=AXIS2_PLACEMENT_3D('',#16307,#13373,#13374);
#11969=AXIS2_PLACEMENT_3D('',#16308,#13375,#13376);
#11970=AXIS2_PLACEMENT_3D('',#16310,#13377,#13378);
#11971=AXIS2_PLACEMENT_3D('',#16312,#13380,#13381);
#11972=AXIS2_PLACEMENT_3D('',#16321,#13386,#13387);
#11973=AXIS2_PLACEMENT_3D('',#16327,#13391,#13392);
#11974=AXIS2_PLACEMENT_3D('',#16333,#13396,#13397);
#11975=AXIS2_PLACEMENT_3D('',#16336,#13400,#13401);
#11976=AXIS2_PLACEMENT_3D('',#16337,#13402,#13403);
#13222=DIRECTION('axis',(0.,0.,1.));
#13223=DIRECTION('refdir',(1.,0.,0.));
#13224=DIRECTION('center_axis',(0.,1.,0.));
#13225=DIRECTION('ref_axis',(1.,0.,0.));
#13226=DIRECTION('center_axis',(0.,1.,0.));
#13227=DIRECTION('ref_axis',(1.,0.,0.));
#13228=DIRECTION('',(0.,1.,0.));
#13229=DIRECTION('center_axis',(0.,-1.,0.));
#13230=DIRECTION('ref_axis',(1.,0.,0.));
#13231=DIRECTION('center_axis',(0.,1.,0.));
#13232=DIRECTION('ref_axis',(1.,0.,0.));
#13233=DIRECTION('center_axis',(0.,1.,0.));
#13234=DIRECTION('ref_axis',(1.,0.,0.));
#13235=DIRECTION('',(0.,1.,0.));
#13236=DIRECTION('center_axis',(0.,-1.,0.));
#13237=DIRECTION('ref_axis',(1.,0.,0.));
#13238=DIRECTION('center_axis',(0.,1.,0.));
#13239=DIRECTION('ref_axis',(1.,0.,0.));
#13240=DIRECTION('center_axis',(0.,1.,0.));
#13241=DIRECTION('ref_axis',(1.,0.,0.));
#13242=DIRECTION('',(0.,1.,0.));
#13243=DIRECTION('center_axis',(0.,-1.,0.));
#13244=DIRECTION('ref_axis',(1.,0.,0.));
#13245=DIRECTION('center_axis',(0.,1.,0.));
#13246=DIRECTION('ref_axis',(1.,0.,0.));
#13247=DIRECTION('center_axis',(0.,1.,0.));
#13248=DIRECTION('ref_axis',(1.,0.,0.));
#13249=DIRECTION('',(0.,1.,0.));
#13250=DIRECTION('center_axis',(0.,-1.,0.));
#13251=DIRECTION('ref_axis',(1.,0.,0.));
#13252=DIRECTION('center_axis',(0.,1.,0.));
#13253=DIRECTION('ref_axis',(1.,0.,0.));
#13254=DIRECTION('center_axis',(0.,1.,0.));
#13255=DIRECTION('ref_axis',(1.,0.,0.));
#13256=DIRECTION('',(0.,1.,0.));
#13257=DIRECTION('center_axis',(0.,-1.,0.));
#13258=DIRECTION('ref_axis',(1.,0.,0.));
#13259=DIRECTION('center_axis',(0.,1.,0.));
#13260=DIRECTION('ref_axis',(1.,0.,0.));
#13261=DIRECTION('center_axis',(0.,1.,0.));
#13262=DIRECTION('ref_axis',(1.,0.,0.));
#13263=DIRECTION('',(0.,1.,0.));
#13264=DIRECTION('center_axis',(0.,-1.,0.));
#13265=DIRECTION('ref_axis',(1.,0.,0.));
#13266=DIRECTION('center_axis',(0.,1.,0.));
#13267=DIRECTION('ref_axis',(1.,0.,0.));
#13268=DIRECTION('center_axis',(0.,1.,0.));
#13269=DIRECTION('ref_axis',(1.,0.,0.));
#13270=DIRECTION('',(0.,1.,0.));
#13271=DIRECTION('center_axis',(0.,-1.,0.));
#13272=DIRECTION('ref_axis',(1.,0.,0.));
#13273=DIRECTION('center_axis',(0.,1.,0.));
#13274=DIRECTION('ref_axis',(1.,0.,0.));
#13275=DIRECTION('center_axis',(0.,1.,0.));
#13276=DIRECTION('ref_axis',(1.,0.,0.));
#13277=DIRECTION('center_axis',(0.,1.,0.));
#13278=DIRECTION('ref_axis',(1.,0.,0.));
#13279=DIRECTION('center_axis',(0.,1.,0.));
#13280=DIRECTION('ref_axis',(1.,0.,0.));
#13281=DIRECTION('',(0.,1.,0.));
#13282=DIRECTION('center_axis',(0.,-1.,0.));
#13283=DIRECTION('ref_axis',(1.,0.,0.));
#13284=DIRECTION('center_axis',(0.,1.,0.));
#13285=DIRECTION('ref_axis',(1.,0.,0.));
#13286=DIRECTION('center_axis',(0.,1.,0.));
#13287=DIRECTION('ref_axis',(1.,0.,0.));
#13288=DIRECTION('center_axis',(0.,1.,0.));
#13289=DIRECTION('ref_axis',(1.,0.,0.));
#13290=DIRECTION('center_axis',(0.,1.,0.));
#13291=DIRECTION('ref_axis',(1.,0.,0.));
#13292=DIRECTION('',(0.,1.,0.));
#13293=DIRECTION('center_axis',(0.,-1.,0.));
#13294=DIRECTION('ref_axis',(1.,0.,0.));
#13295=DIRECTION('center_axis',(0.,1.,0.));
#13296=DIRECTION('ref_axis',(1.,0.,0.));
#13297=DIRECTION('center_axis',(0.,1.,0.));
#13298=DIRECTION('ref_axis',(1.,0.,0.));
#13299=DIRECTION('center_axis',(0.,1.,0.));
#13300=DIRECTION('ref_axis',(1.,0.,0.));
#13301=DIRECTION('center_axis',(0.,1.,0.));
#13302=DIRECTION('ref_axis',(1.,0.,0.));
#13303=DIRECTION('',(0.,1.,0.));
#13304=DIRECTION('center_axis',(0.,-1.,0.));
#13305=DIRECTION('ref_axis',(1.,0.,0.));
#13306=DIRECTION('center_axis',(0.,1.,0.));
#13307=DIRECTION('ref_axis',(1.,0.,0.));
#13308=DIRECTION('center_axis',(0.,1.,0.));
#13309=DIRECTION('ref_axis',(1.,0.,0.));
#13310=DIRECTION('center_axis',(0.,1.,0.));
#13311=DIRECTION('ref_axis',(1.,0.,0.));
#13312=DIRECTION('center_axis',(0.,1.,0.));
#13313=DIRECTION('ref_axis',(1.,0.,0.));
#13314=DIRECTION('',(0.,1.,0.));
#13315=DIRECTION('center_axis',(0.,1.,0.));
#13316=DIRECTION('ref_axis',(1.,0.,0.));
#13317=DIRECTION('center_axis',(0.,1.,0.));
#13318=DIRECTION('ref_axis',(1.,0.,0.));
#13319=DIRECTION('',(0.,1.,0.));
#13320=DIRECTION('center_axis',(0.,1.,0.));
#13321=DIRECTION('ref_axis',(1.,0.,0.));
#13322=DIRECTION('center_axis',(0.,1.,0.));
#13323=DIRECTION('ref_axis',(1.,0.,0.));
#13324=DIRECTION('',(0.,1.,0.));
#13325=DIRECTION('center_axis',(0.,1.,0.));
#13326=DIRECTION('ref_axis',(1.,0.,0.));
#13327=DIRECTION('center_axis',(0.,1.,0.));
#13328=DIRECTION('ref_axis',(1.,0.,0.));
#13329=DIRECTION('',(0.,1.,0.));
#13330=DIRECTION('center_axis',(0.,0.,1.));
#13331=DIRECTION('ref_axis',(1.,0.,0.));
#13332=DIRECTION('center_axis',(0.,0.,1.));
#13333=DIRECTION('ref_axis',(1.,0.,0.));
#13334=DIRECTION('',(0.,0.,1.));
#13335=DIRECTION('center_axis',(0.,0.,1.));
#13336=DIRECTION('ref_axis',(1.,0.,0.));
#13337=DIRECTION('center_axis',(0.,0.,1.));
#13338=DIRECTION('ref_axis',(1.,0.,0.));
#13339=DIRECTION('center_axis',(0.,0.,1.));
#13340=DIRECTION('ref_axis',(1.,0.,0.));
#13341=DIRECTION('center_axis',(0.,0.,1.));
#13342=DIRECTION('ref_axis',(1.,0.,0.));
#13343=DIRECTION('',(0.,0.,1.));
#13344=DIRECTION('center_axis',(0.,0.,1.));
#13345=DIRECTION('ref_axis',(1.,0.,0.));
#13346=DIRECTION('center_axis',(0.,0.,1.));
#13347=DIRECTION('ref_axis',(1.,0.,0.));
#13348=DIRECTION('center_axis',(0.,1.,0.));
#13349=DIRECTION('ref_axis',(1.,0.,0.));
#13350=DIRECTION('center_axis',(0.,1.,0.));
#13351=DIRECTION('ref_axis',(1.,0.,0.));
#13352=DIRECTION('',(0.,1.,0.));
#13353=DIRECTION('center_axis',(0.,-1.,0.));
#13354=DIRECTION('ref_axis',(1.,0.,0.));
#13355=DIRECTION('center_axis',(0.,1.,0.));
#13356=DIRECTION('ref_axis',(1.,0.,0.));
#13357=DIRECTION('center_axis',(0.,1.,0.));
#13358=DIRECTION('ref_axis',(1.,0.,0.));
#13359=DIRECTION('center_axis',(0.,1.,0.));
#13360=DIRECTION('ref_axis',(1.,0.,0.));
#13361=DIRECTION('center_axis',(0.,1.,0.));
#13362=DIRECTION('ref_axis',(1.,0.,0.));
#13363=DIRECTION('',(0.,1.,0.));
#13364=DIRECTION('center_axis',(0.,1.,0.));
#13365=DIRECTION('ref_axis',(1.,0.,0.));
#13366=DIRECTION('center_axis',(0.,1.,0.));
#13367=DIRECTION('ref_axis',(1.,0.,0.));
#13368=DIRECTION('',(0.,1.,0.));
#13369=DIRECTION('center_axis',(0.,-1.,0.));
#13370=DIRECTION('ref_axis',(1.,0.,0.));
#13371=DIRECTION('center_axis',(0.,1.,0.));
#13372=DIRECTION('ref_axis',(1.,0.,0.));
#13373=DIRECTION('center_axis',(0.,1.,0.));
#13374=DIRECTION('ref_axis',(1.,0.,0.));
#13375=DIRECTION('center_axis',(0.,1.,0.));
#13376=DIRECTION('ref_axis',(1.,0.,0.));
#13377=DIRECTION('center_axis',(0.,1.,0.));
#13378=DIRECTION('ref_axis',(1.,0.,0.));
#13379=DIRECTION('',(0.,1.,0.));
#13380=DIRECTION('center_axis',(0.,1.,0.));
#13381=DIRECTION('ref_axis',(-1.,0.,0.));
#13382=DIRECTION('',(-1.,0.,0.));
#13383=DIRECTION('',(0.,0.,1.));
#13384=DIRECTION('',(-1.,0.,0.));
#13385=DIRECTION('',(0.,0.,1.));
#13386=DIRECTION('center_axis',(1.,0.,0.));
#13387=DIRECTION('ref_axis',(0.,1.,0.));
#13388=DIRECTION('',(0.,1.,0.));
#13389=DIRECTION('',(0.,1.,0.));
#13390=DIRECTION('',(0.,0.,1.));
#13391=DIRECTION('center_axis',(0.,-1.,0.));
#13392=DIRECTION('ref_axis',(1.,0.,0.));
#13393=DIRECTION('',(1.,0.,0.));
#13394=DIRECTION('',(1.,0.,0.));
#13395=DIRECTION('',(0.,0.,1.));
#13396=DIRECTION('center_axis',(-1.,0.,0.));
#13397=DIRECTION('ref_axis',(0.,-1.,0.));
#13398=DIRECTION('',(0.,-1.,0.));
#13399=DIRECTION('',(0.,-1.,0.));
#13400=DIRECTION('center_axis',(0.,0.,1.));
#13401=DIRECTION('ref_axis',(1.,0.,0.));
#13402=DIRECTION('center_axis',(0.,0.,1.));
#13403=DIRECTION('ref_axis',(1.,0.,0.));
#16183=CARTESIAN_POINT('',(0.,0.,0.));
#16184=CARTESIAN_POINT('Origin',(6.,2.5,7.6));
#16185=CARTESIAN_POINT('',(5.835,2.6,7.6));
#16186=CARTESIAN_POINT('Origin',(6.,2.6,7.6));
#16187=CARTESIAN_POINT('',(5.835,4.4,7.6));
#16188=CARTESIAN_POINT('',(5.835,2.5,7.6));
#16189=CARTESIAN_POINT('Origin',(6.,4.4,7.6));
#16190=CARTESIAN_POINT('Origin',(3.74833395016046,2.5,3.7));
#16191=CARTESIAN_POINT('',(3.58333395016046,2.6,3.7));
#16192=CARTESIAN_POINT('Origin',(3.74833395016046,2.6,3.7));
#16193=CARTESIAN_POINT('',(3.58333395016046,4.4,3.7));
#16194=CARTESIAN_POINT('',(3.58333395016046,2.5,3.7));
#16195=CARTESIAN_POINT('Origin',(3.74833395016046,4.4,3.7));
#16196=CARTESIAN_POINT('Origin',(8.25166604983954,2.5,3.7));
#16197=CARTESIAN_POINT('',(8.08666604983954,2.6,3.7));
#16198=CARTESIAN_POINT('Origin',(8.25166604983954,2.6,3.7));
#16199=CARTESIAN_POINT('',(8.08666604983954,4.4,3.7));
#16200=CARTESIAN_POINT('',(8.08666604983954,2.5,3.7));
#16201=CARTESIAN_POINT('Origin',(8.25166604983954,4.4,3.7));
#16202=CARTESIAN_POINT('Origin',(1.16341445918999E-16,2.5,6.9));
#16203=CARTESIAN_POINT('',(-0.165,2.6,6.9));
#16204=CARTESIAN_POINT('Origin',(1.16341445918999E-16,2.6,6.9));
#16205=CARTESIAN_POINT('',(-0.165,4.4,6.9));
#16206=CARTESIAN_POINT('',(-0.165,2.5,6.9));
#16207=CARTESIAN_POINT('Origin',(1.16341445918999E-16,4.4,6.9));
#16208=CARTESIAN_POINT('Origin',(-1.64544826719043,2.5,4.05));
#16209=CARTESIAN_POINT('',(-1.81044826719043,2.6,4.05));
#16210=CARTESIAN_POINT('Origin',(-1.64544826719043,2.6,4.05));
#16211=CARTESIAN_POINT('',(-1.81044826719043,4.4,4.05));
#16212=CARTESIAN_POINT('',(-1.81044826719043,2.5,4.05));
#16213=CARTESIAN_POINT('Origin',(-1.64544826719043,4.4,4.05));
#16214=CARTESIAN_POINT('Origin',(1.64544826719043,2.5,4.05));
#16215=CARTESIAN_POINT('',(1.48044826719043,2.6,4.05));
#16216=CARTESIAN_POINT('Origin',(1.64544826719043,2.6,4.05));
#16217=CARTESIAN_POINT('',(1.48044826719043,4.4,4.05));
#16218=CARTESIAN_POINT('',(1.48044826719043,2.5,4.05));
#16219=CARTESIAN_POINT('Origin',(1.64544826719043,4.4,4.05));
#16220=CARTESIAN_POINT('Origin',(10.,3.9,2.));
#16221=CARTESIAN_POINT('',(9.525,3.9,2.));
#16222=CARTESIAN_POINT('Origin',(10.,3.9,2.));
#16223=CARTESIAN_POINT('',(9.525,4.4,2.));
#16224=CARTESIAN_POINT('',(9.525,3.9,2.));
#16225=CARTESIAN_POINT('Origin',(10.,4.4,2.));
#16226=CARTESIAN_POINT('Origin',(10.,3.9,2.));
#16227=CARTESIAN_POINT('',(9.725,3.9,2.));
#16228=CARTESIAN_POINT('Origin',(10.,3.9,2.));
#16229=CARTESIAN_POINT('Origin',(-2.,3.9,9.));
#16230=CARTESIAN_POINT('',(-2.475,3.9,9.));
#16231=CARTESIAN_POINT('Origin',(-2.,3.9,9.));
#16232=CARTESIAN_POINT('',(-2.475,4.4,9.));
#16233=CARTESIAN_POINT('',(-2.475,3.9,9.));
#16234=CARTESIAN_POINT('Origin',(-2.,4.4,9.));
#16235=CARTESIAN_POINT('Origin',(-2.,3.9,9.));
#16236=CARTESIAN_POINT('',(-2.275,3.9,9.));
#16237=CARTESIAN_POINT('Origin',(-2.,3.9,9.));
#16238=CARTESIAN_POINT('Origin',(-2.,3.9,2.));
#16239=CARTESIAN_POINT('',(-2.475,3.9,2.));
#16240=CARTESIAN_POINT('Origin',(-2.,3.9,2.));
#16241=CARTESIAN_POINT('',(-2.475,4.4,2.));
#16242=CARTESIAN_POINT('',(-2.475,3.9,2.));
#16243=CARTESIAN_POINT('Origin',(-2.,4.4,2.));
#16244=CARTESIAN_POINT('Origin',(-2.,3.9,2.));
#16245=CARTESIAN_POINT('',(-2.275,3.9,2.));
#16246=CARTESIAN_POINT('Origin',(-2.,3.9,2.));
#16247=CARTESIAN_POINT('Origin',(10.,3.9,9.));
#16248=CARTESIAN_POINT('',(9.525,3.9,9.));
#16249=CARTESIAN_POINT('Origin',(10.,3.9,9.));
#16250=CARTESIAN_POINT('',(9.525,4.4,9.));
#16251=CARTESIAN_POINT('',(9.525,3.9,9.));
#16252=CARTESIAN_POINT('Origin',(10.,4.4,9.));
#16253=CARTESIAN_POINT('Origin',(10.,3.9,9.));
#16254=CARTESIAN_POINT('',(9.725,3.9,9.));
#16255=CARTESIAN_POINT('Origin',(10.,3.9,9.));
#16256=CARTESIAN_POINT('Origin',(10.,2.5,2.));
#16257=CARTESIAN_POINT('',(9.725,2.6,2.));
#16258=CARTESIAN_POINT('Origin',(10.,2.6,2.));
#16259=CARTESIAN_POINT('',(9.725,2.5,2.));
#16260=CARTESIAN_POINT('Origin',(-2.,2.5,9.));
#16261=CARTESIAN_POINT('',(-2.275,2.6,9.));
#16262=CARTESIAN_POINT('Origin',(-2.,2.6,9.));
#16263=CARTESIAN_POINT('',(-2.275,2.5,9.));
#16264=CARTESIAN_POINT('Origin',(-2.,2.5,2.));
#16265=CARTESIAN_POINT('',(-2.275,2.6,2.));
#16266=CARTESIAN_POINT('Origin',(-2.,2.6,2.));
#16267=CARTESIAN_POINT('',(-2.275,2.5,2.));
#16268=CARTESIAN_POINT('Origin',(10.,2.5,9.));
#16269=CARTESIAN_POINT('',(9.725,2.6,9.));
#16270=CARTESIAN_POINT('Origin',(10.,2.6,9.));
#16271=CARTESIAN_POINT('',(9.725,2.5,9.));
#16272=CARTESIAN_POINT('Origin',(10.,3.5,-0.1));
#16273=CARTESIAN_POINT('',(9.75,3.5,0.));
#16274=CARTESIAN_POINT('Origin',(10.,3.5,0.));
#16275=CARTESIAN_POINT('',(9.75,3.5,1.7));
#16276=CARTESIAN_POINT('',(9.75,3.5,-0.1));
#16277=CARTESIAN_POINT('Origin',(10.,3.5,1.7));
#16278=CARTESIAN_POINT('Origin',(10.,3.5,1.7));
#16279=CARTESIAN_POINT('Origin',(-2.,3.5,-0.1));
#16280=CARTESIAN_POINT('',(-2.25,3.5,0.));
#16281=CARTESIAN_POINT('Origin',(-2.,3.5,0.));
#16282=CARTESIAN_POINT('',(-2.25,3.5,1.7));
#16283=CARTESIAN_POINT('',(-2.25,3.5,-0.1));
#16284=CARTESIAN_POINT('Origin',(-2.,3.5,1.7));
#16285=CARTESIAN_POINT('Origin',(-2.,3.5,1.7));
#16286=CARTESIAN_POINT('Origin',(6.,2.8,5.));
#16287=CARTESIAN_POINT('',(3.65,2.8,5.));
#16288=CARTESIAN_POINT('Origin',(6.,2.8,5.));
#16289=CARTESIAN_POINT('',(3.65,4.4,5.));
#16290=CARTESIAN_POINT('',(3.65,2.8,5.));
#16291=CARTESIAN_POINT('Origin',(6.,4.4,5.));
#16292=CARTESIAN_POINT('Origin',(6.,2.8,5.));
#16293=CARTESIAN_POINT('',(3.85,2.8,5.));
#16294=CARTESIAN_POINT('Origin',(6.,2.8,5.));
#16295=CARTESIAN_POINT('Origin',(6.,2.5,5.));
#16296=CARTESIAN_POINT('',(3.85,2.6,5.));
#16297=CARTESIAN_POINT('Origin',(6.,2.6,5.));
#16298=CARTESIAN_POINT('',(3.85,2.5,5.));
#16299=CARTESIAN_POINT('Origin',(0.,3.,5.));
#16300=CARTESIAN_POINT('',(-1.6,3.,5.));
#16301=CARTESIAN_POINT('Origin',(0.,3.,5.));
#16302=CARTESIAN_POINT('',(-1.6,4.4,5.));
#16303=CARTESIAN_POINT('',(-1.6,3.,5.));
#16304=CARTESIAN_POINT('Origin',(0.,4.4,5.));
#16305=CARTESIAN_POINT('Origin',(0.,3.,5.));
#16306=CARTESIAN_POINT('',(-1.4,3.,5.));
#16307=CARTESIAN_POINT('Origin',(0.,3.,5.));
#16308=CARTESIAN_POINT('Origin',(0.,2.5,5.));
#16309=CARTESIAN_POINT('',(-1.4,2.6,5.));
#16310=CARTESIAN_POINT('Origin',(0.,2.6,5.));
#16311=CARTESIAN_POINT('',(-1.4,2.5,5.));
#16312=CARTESIAN_POINT('Origin',(11.,4.4,0.));
#16313=CARTESIAN_POINT('',(11.,4.4,0.));
#16314=CARTESIAN_POINT('',(-3.,4.4,0.));
#16315=CARTESIAN_POINT('',(11.,4.4,0.));
#16316=CARTESIAN_POINT('',(-3.,4.4,10.));
#16317=CARTESIAN_POINT('',(-3.,4.4,0.));
#16318=CARTESIAN_POINT('',(11.,4.4,10.));
#16319=CARTESIAN_POINT('',(11.,4.4,10.));
#16320=CARTESIAN_POINT('',(11.,4.4,0.));
#16321=CARTESIAN_POINT('Origin',(11.,2.6,0.));
#16322=CARTESIAN_POINT('',(11.,2.6,0.));
#16323=CARTESIAN_POINT('',(11.,2.6,0.));
#16324=CARTESIAN_POINT('',(11.,2.6,10.));
#16325=CARTESIAN_POINT('',(11.,2.6,10.));
#16326=CARTESIAN_POINT('',(11.,2.6,0.));
#16327=CARTESIAN_POINT('Origin',(-3.,2.6,0.));
#16328=CARTESIAN_POINT('',(-3.,2.6,0.));
#16329=CARTESIAN_POINT('',(-3.,2.6,0.));
#16330=CARTESIAN_POINT('',(-3.,2.6,10.));
#16331=CARTESIAN_POINT('',(-3.,2.6,10.));
#16332=CARTESIAN_POINT('',(-3.,2.6,0.));
#16333=CARTESIAN_POINT('Origin',(-3.,4.4,0.));
#16334=CARTESIAN_POINT('',(-3.,4.4,0.));
#16335=CARTESIAN_POINT('',(-3.,4.4,10.));
#16336=CARTESIAN_POINT('Origin',(4.,3.5,10.));
#16337=CARTESIAN_POINT('Origin',(4.,3.5,0.));
#53814=UNCERTAINTY_MEASURE_WITH_UNIT(LENGTH_MEASURE(0.001),#53910,
'DISTANCE_ACCURACY_VALUE',
'Maximum model space distance between geometric entities at asserted c
onnectivities');
#53859=UNCERTAINTY_MEASURE_WITH_UNIT(LENGTH_MEASURE(0.001),#53910,
'DISTANCE_ACCURACY_VALUE',
'Maximum model space distance between geometric entities at asserted c
onnectivities');
#53864=(
GEOMETRIC_REPRESENTATION_CONTEXT(3)
GLOBAL_UNCERTAINTY_ASSIGNED_CONTEXT((#53814))
GLOBAL_UNIT_ASSIGNED_CONTEXT((#53910,#53912,#53913))
REPRESENTATION_CONTEXT('','3D')
);
#53909=(
GEOMETRIC_REPRESENTATION_CONTEXT(3)
GLOBAL_UNCERTAINTY_ASSIGNED_CONTEXT((#53859))
GLOBAL_UNIT_ASSIGNED_CONTEXT((#53910,#53912,#53913))
REPRESENTATION_CONTEXT('','3D')
);
#53910=(
LENGTH_UNIT()
NAMED_UNIT(*)
SI_UNIT(.CENTI.,.METRE.)
);
#53912=(
NAMED_UNIT(*)
PLANE_ANGLE_UNIT()
SI_UNIT($,.RADIAN.)
);
#53913=(
NAMED_UNIT(*)
SI_UNIT($,.STERADIAN.)
SOLID_ANGLE_UNIT()
);
#53918=SHAPE_DEFINITION_REPRESENTATION(#53967,#54090);
#53967=PRODUCT_DEFINITION_SHAPE('',$,#54140);
#54090=SHAPE_REPRESENTATION('',(#11902),#53864);
#54135=PRODUCT_DEFINITION_CONTEXT('part definition',#54284,'design');
#54140=PRODUCT_DEFINITION('Rear plate','Rear plate',#54189,#54135);
#54189=PRODUCT_DEFINITION_FORMATION('',$,#54290);
#54284=APPLICATION_CONTEXT(
'Core Data for Automotive Mechanical Design Process');
#54285=PRODUCT_CONTEXT('part definition',#54284,'mechanical');
#54290=PRODUCT('Rear plate','Rear plate','Rear plate',(#54285));
#54405=COLOUR_RGB('Off White',0.89,0.88,0.83);
#54406=FILL_AREA_STYLE_COLOUR('',#54405);
#54407=FILL_AREA_STYLE('',(#54406));
#54408=SURFACE_STYLE_FILL_AREA(#54407);
#54409=SURFACE_SIDE_STYLE('',(#54408));
#54410=SURFACE_STYLE_USAGE(.BOTH.,#54409);
#54411=PRESENTATION_STYLE_ASSIGNMENT((#54410));
ENDSEC;
END-ISO-10303-21;
